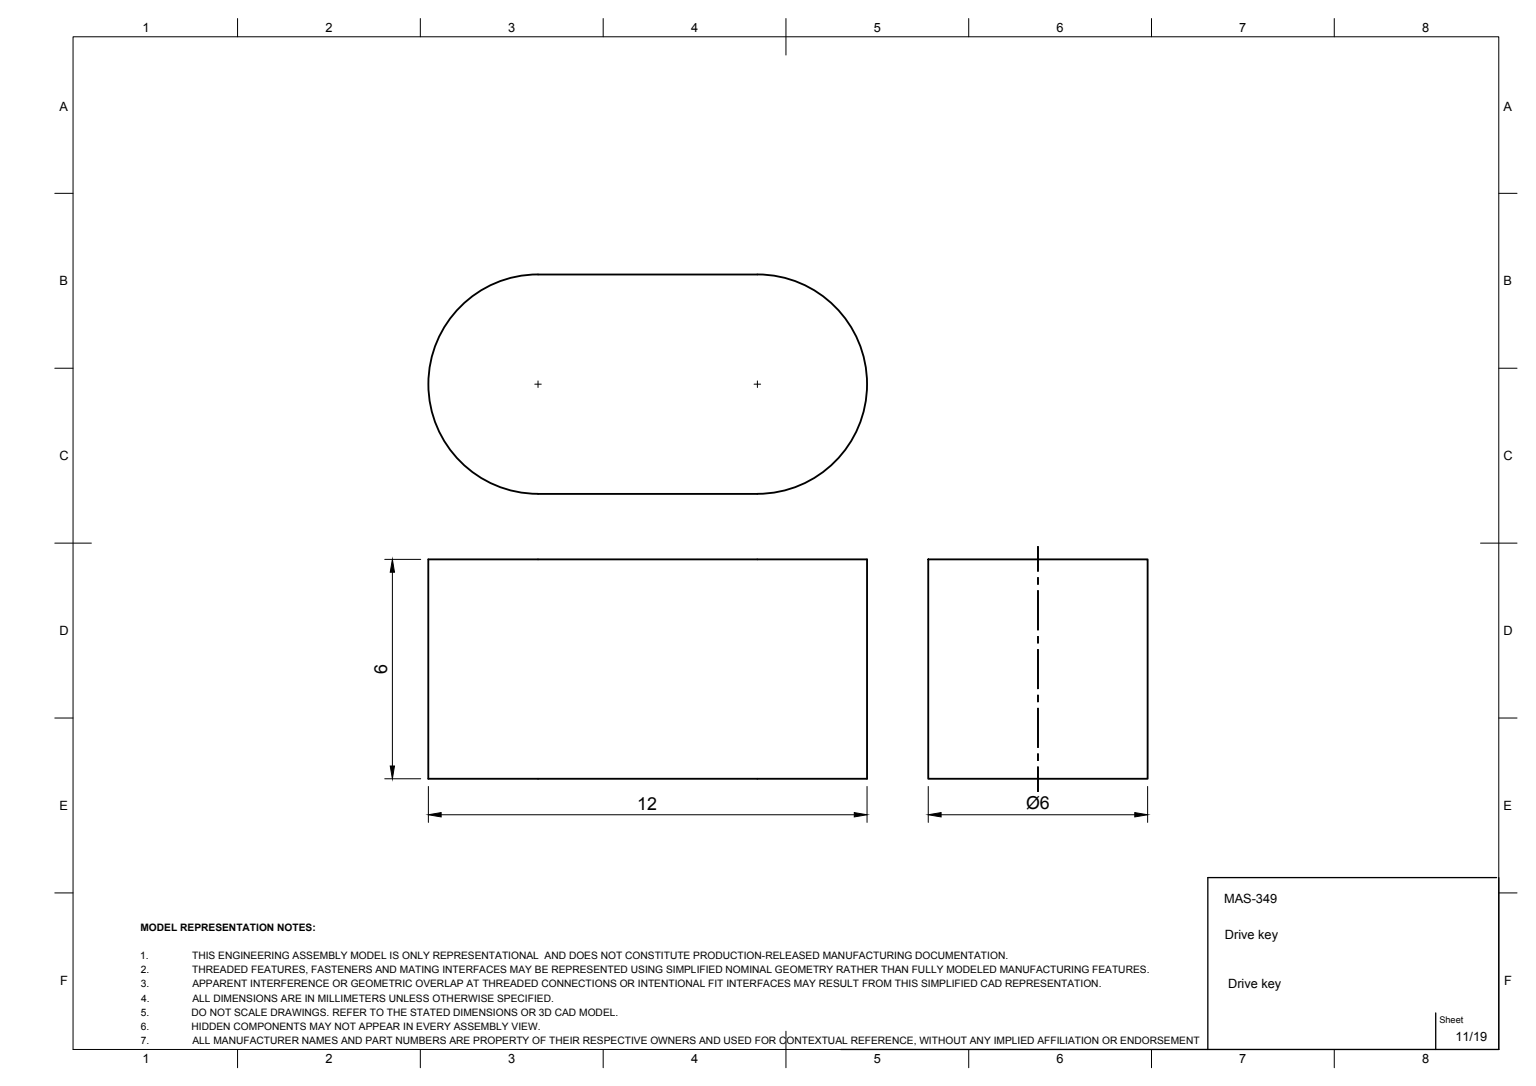
ISO-10303-21;
HEADER;
/* Generated by software containing ST-Developer
 * from STEP Tools, Inc. (www.steptools.com) 
 */

FILE_DESCRIPTION(
/* description */ ('Independent two-stage semi-open centrifugal-pump CAD. Shared impeller
s, open-machinable return casings, removable diaphragms, bronze wear/j
ournal rings, volume-preserving seal instances, retained keyed shaft, 
opposed mechanical face rings and partly threaded tie hardware. Native
 shaft rotation. Geometric topology/clearance only; flow/head/efficien
cy, pressure, cavitation, balance, preload, face loading and secondary
 seal fits/bonds, material/thermal/tolerance selection and life unassi
gned. External drive, coupling, anchors and piping bolts omitted.'),
/* implementation_level */ '2;1');

FILE_NAME(
/* name */ 'Drive key.step',
/* time_stamp */ '2026-11-08T18:06:32-08:00',
/* author */ (''),
/* organization */ (''),
/* preprocessor_version */ 'ST-DEVELOPER v20.2',
/* originating_system */ 'Autodesk Translation Framework v15.17.0.0',
/* authorisation */ '');

FILE_SCHEMA (('AUTOMOTIVE_DESIGN { 1 0 10303 214 3 1 1 }'));
ENDSEC;

DATA;
#10=MECHANICAL_DESIGN_GEOMETRIC_PRESENTATION_REPRESENTATION('',(#405),#16687);
#367=SHAPE_REPRESENTATION_RELATIONSHIP('SRR','None',#16776,#386);
#386=ADVANCED_BREP_SHAPE_REPRESENTATION('',(#424),#16680);
#405=STYLED_ITEM('',(#16876),#424);
#424=MANIFOLD_SOLID_BREP('Body1',#6124);
#659=PLANE('',#6861);
#660=PLANE('',#6865);
#661=PLANE('',#6869);
#662=PLANE('',#6870);
#974=FACE_OUTER_BOUND('',#1433,.T.);
#975=FACE_OUTER_BOUND('',#1434,.T.);
#976=FACE_OUTER_BOUND('',#1435,.T.);
#977=FACE_OUTER_BOUND('',#1436,.T.);
#978=FACE_OUTER_BOUND('',#1437,.T.);
#979=FACE_OUTER_BOUND('',#1438,.T.);
#1433=EDGE_LOOP('',(#5305,#5306,#5307,#5308));
#1434=EDGE_LOOP('',(#5309,#5310,#5311,#5312));
#1435=EDGE_LOOP('',(#5313,#5314,#5315,#5316));
#1436=EDGE_LOOP('',(#5317,#5318,#5319,#5320));
#1437=EDGE_LOOP('',(#5321,#5322,#5323,#5324));
#1438=EDGE_LOOP('',(#5325,#5326,#5327,#5328));
#1812=LINE('',#15164,#2181);
#1813=LINE('',#15166,#2182);
#1814=LINE('',#15168,#2183);
#1815=LINE('',#15169,#2184);
#1816=LINE('',#15175,#2185);
#1817=LINE('',#15178,#2186);
#1818=LINE('',#15180,#2187);
#1819=LINE('',#15181,#2188);
#2181=VECTOR('',#8340,1.);
#2182=VECTOR('',#8341,1.);
#2183=VECTOR('',#8342,1.);
#2184=VECTOR('',#8343,1.);
#2185=VECTOR('',#8350,1.);
#2186=VECTOR('',#8353,1.);
#2187=VECTOR('',#8354,1.);
#2188=VECTOR('',#8355,1.);
#2466=CIRCLE('',#6863,0.3);
#2467=CIRCLE('',#6864,0.3);
#2468=CIRCLE('',#6867,0.3);
#2469=CIRCLE('',#6868,0.3);
#2969=VERTEX_POINT('',#15162);
#2970=VERTEX_POINT('',#15163);
#2971=VERTEX_POINT('',#15165);
#2972=VERTEX_POINT('',#15167);
#2973=VERTEX_POINT('',#15171);
#2974=VERTEX_POINT('',#15173);
#2975=VERTEX_POINT('',#15177);
#2976=VERTEX_POINT('',#15179);
#3762=EDGE_CURVE('',#2969,#2970,#1812,.T.);
#3763=EDGE_CURVE('',#2969,#2971,#1813,.T.);
#3764=EDGE_CURVE('',#2972,#2971,#1814,.T.);
#3765=EDGE_CURVE('',#2970,#2972,#1815,.T.);
#3766=EDGE_CURVE('',#2973,#2970,#2466,.T.);
#3767=EDGE_CURVE('',#2974,#2972,#2467,.T.);
#3768=EDGE_CURVE('',#2973,#2974,#1816,.T.);
#3769=EDGE_CURVE('',#2973,#2975,#1817,.T.);
#3770=EDGE_CURVE('',#2976,#2974,#1818,.T.);
#3771=EDGE_CURVE('',#2975,#2976,#1819,.T.);
#3772=EDGE_CURVE('',#2969,#2975,#2468,.T.);
#3773=EDGE_CURVE('',#2971,#2976,#2469,.T.);
#5305=ORIENTED_EDGE('',*,*,#3762,.F.);
#5306=ORIENTED_EDGE('',*,*,#3763,.T.);
#5307=ORIENTED_EDGE('',*,*,#3764,.F.);
#5308=ORIENTED_EDGE('',*,*,#3765,.F.);
#5309=ORIENTED_EDGE('',*,*,#3766,.T.);
#5310=ORIENTED_EDGE('',*,*,#3765,.T.);
#5311=ORIENTED_EDGE('',*,*,#3767,.F.);
#5312=ORIENTED_EDGE('',*,*,#3768,.F.);
#5313=ORIENTED_EDGE('',*,*,#3769,.F.);
#5314=ORIENTED_EDGE('',*,*,#3768,.T.);
#5315=ORIENTED_EDGE('',*,*,#3770,.F.);
#5316=ORIENTED_EDGE('',*,*,#3771,.F.);
#5317=ORIENTED_EDGE('',*,*,#3772,.T.);
#5318=ORIENTED_EDGE('',*,*,#3771,.T.);
#5319=ORIENTED_EDGE('',*,*,#3773,.F.);
#5320=ORIENTED_EDGE('',*,*,#3763,.F.);
#5321=ORIENTED_EDGE('',*,*,#3773,.T.);
#5322=ORIENTED_EDGE('',*,*,#3770,.T.);
#5323=ORIENTED_EDGE('',*,*,#3767,.T.);
#5324=ORIENTED_EDGE('',*,*,#3764,.T.);
#5325=ORIENTED_EDGE('',*,*,#3772,.F.);
#5326=ORIENTED_EDGE('',*,*,#3762,.T.);
#5327=ORIENTED_EDGE('',*,*,#3766,.F.);
#5328=ORIENTED_EDGE('',*,*,#3769,.T.);
#5736=CYLINDRICAL_SURFACE('',#6862,0.3);
#5737=CYLINDRICAL_SURFACE('',#6866,0.3);
#6053=ADVANCED_FACE('',(#974),#659,.T.);
#6054=ADVANCED_FACE('',(#975),#5736,.T.);
#6055=ADVANCED_FACE('',(#976),#660,.T.);
#6056=ADVANCED_FACE('',(#977),#5737,.T.);
#6057=ADVANCED_FACE('',(#978),#661,.T.);
#6058=ADVANCED_FACE('',(#979),#662,.F.);
#6124=CLOSED_SHELL('',(#6053,#6054,#6055,#6056,#6057,#6058));
#6860=AXIS2_PLACEMENT_3D('',#15160,#8336,#8337);
#6861=AXIS2_PLACEMENT_3D('',#15161,#8338,#8339);
#6862=AXIS2_PLACEMENT_3D('',#15170,#8344,#8345);
#6863=AXIS2_PLACEMENT_3D('',#15172,#8346,#8347);
#6864=AXIS2_PLACEMENT_3D('',#15174,#8348,#8349);
#6865=AXIS2_PLACEMENT_3D('',#15176,#8351,#8352);
#6866=AXIS2_PLACEMENT_3D('',#15182,#8356,#8357);
#6867=AXIS2_PLACEMENT_3D('',#15183,#8358,#8359);
#6868=AXIS2_PLACEMENT_3D('',#15184,#8360,#8361);
#6869=AXIS2_PLACEMENT_3D('',#15185,#8362,#8363);
#6870=AXIS2_PLACEMENT_3D('',#15186,#8364,#8365);
#8336=DIRECTION('axis',(0.,0.,1.));
#8337=DIRECTION('refdir',(1.,0.,0.));
#8338=DIRECTION('center_axis',(0.,1.,0.));
#8339=DIRECTION('ref_axis',(0.,0.,1.));
#8340=DIRECTION('',(0.,0.,-1.));
#8341=DIRECTION('',(1.,0.,0.));
#8342=DIRECTION('',(0.,0.,1.));
#8343=DIRECTION('',(1.,0.,0.));
#8344=DIRECTION('center_axis',(1.,0.,0.));
#8345=DIRECTION('ref_axis',(0.,-1.,0.));
#8346=DIRECTION('center_axis',(1.,0.,0.));
#8347=DIRECTION('ref_axis',(0.,-1.,0.));
#8348=DIRECTION('center_axis',(1.,0.,0.));
#8349=DIRECTION('ref_axis',(0.,-1.,0.));
#8350=DIRECTION('',(1.,0.,0.));
#8351=DIRECTION('center_axis',(0.,-1.,0.));
#8352=DIRECTION('ref_axis',(0.,0.,-1.));
#8353=DIRECTION('',(0.,0.,1.));
#8354=DIRECTION('',(0.,0.,-1.));
#8355=DIRECTION('',(1.,0.,0.));
#8356=DIRECTION('center_axis',(1.,0.,0.));
#8357=DIRECTION('ref_axis',(0.,1.,0.));
#8358=DIRECTION('center_axis',(1.,0.,0.));
#8359=DIRECTION('ref_axis',(0.,1.,0.));
#8360=DIRECTION('center_axis',(1.,0.,0.));
#8361=DIRECTION('ref_axis',(0.,1.,0.));
#8362=DIRECTION('center_axis',(1.,0.,0.));
#8363=DIRECTION('ref_axis',(0.,0.,-1.));
#8364=DIRECTION('center_axis',(1.,0.,0.));
#8365=DIRECTION('ref_axis',(0.,0.,-1.));
#15160=CARTESIAN_POINT('',(0.,0.,0.));
#15161=CARTESIAN_POINT('Origin',(0.,0.3,2.1));
#15162=CARTESIAN_POINT('',(0.,0.3,2.7));
#15163=CARTESIAN_POINT('',(0.,0.3,2.1));
#15164=CARTESIAN_POINT('',(0.,0.3,2.7));
#15165=CARTESIAN_POINT('',(0.6,0.3,2.7));
#15166=CARTESIAN_POINT('',(0.,0.3,2.7));
#15167=CARTESIAN_POINT('',(0.6,0.3,2.1));
#15168=CARTESIAN_POINT('',(0.6,0.3,2.7));
#15169=CARTESIAN_POINT('',(0.,0.3,2.1));
#15170=CARTESIAN_POINT('Origin',(0.,0.,2.1));
#15171=CARTESIAN_POINT('',(0.,-0.3,2.1));
#15172=CARTESIAN_POINT('Origin',(0.,0.,2.1));
#15173=CARTESIAN_POINT('',(0.6,-0.3,2.1));
#15174=CARTESIAN_POINT('Origin',(0.6,0.,2.1));
#15175=CARTESIAN_POINT('',(0.,-0.3,2.1));
#15176=CARTESIAN_POINT('Origin',(0.,-0.3,2.7));
#15177=CARTESIAN_POINT('',(0.,-0.3,2.7));
#15178=CARTESIAN_POINT('',(0.,-0.3,2.1));
#15179=CARTESIAN_POINT('',(0.6,-0.3,2.7));
#15180=CARTESIAN_POINT('',(0.6,-0.3,2.1));
#15181=CARTESIAN_POINT('',(0.,-0.3,2.7));
#15182=CARTESIAN_POINT('Origin',(0.,2.77555756156289E-17,2.7));
#15183=CARTESIAN_POINT('Origin',(0.,2.77555756156289E-17,2.7));
#15184=CARTESIAN_POINT('Origin',(0.6,2.77555756156289E-17,2.7));
#15185=CARTESIAN_POINT('Origin',(0.6,0.,2.4));
#15186=CARTESIAN_POINT('Origin',(0.,0.,2.4));
#16659=UNCERTAINTY_MEASURE_WITH_UNIT(LENGTH_MEASURE(0.001),#16688,
'DISTANCE_ACCURACY_VALUE',
'Maximum model space distance between geometric entities at asserted c
onnectivities');
#16666=UNCERTAINTY_MEASURE_WITH_UNIT(LENGTH_MEASURE(0.001),#16688,
'DISTANCE_ACCURACY_VALUE',
'Maximum model space distance between geometric entities at asserted c
onnectivities');
#16680=(
GEOMETRIC_REPRESENTATION_CONTEXT(3)
GLOBAL_UNCERTAINTY_ASSIGNED_CONTEXT((#16659))
GLOBAL_UNIT_ASSIGNED_CONTEXT((#16688,#16690,#16691))
REPRESENTATION_CONTEXT('','3D')
);
#16687=(
GEOMETRIC_REPRESENTATION_CONTEXT(3)
GLOBAL_UNCERTAINTY_ASSIGNED_CONTEXT((#16666))
GLOBAL_UNIT_ASSIGNED_CONTEXT((#16688,#16690,#16691))
REPRESENTATION_CONTEXT('','3D')
);
#16688=(
LENGTH_UNIT()
NAMED_UNIT(*)
SI_UNIT(.CENTI.,.METRE.)
);
#16690=(
NAMED_UNIT(*)
PLANE_ANGLE_UNIT()
SI_UNIT($,.RADIAN.)
);
#16691=(
NAMED_UNIT(*)
SI_UNIT($,.STERADIAN.)
SOLID_ANGLE_UNIT()
);
#16705=SHAPE_DEFINITION_REPRESENTATION(#16725,#16776);
#16725=PRODUCT_DEFINITION_SHAPE('',$,#16797);
#16776=SHAPE_REPRESENTATION('',(#6860),#16680);
#16783=PRODUCT_DEFINITION_CONTEXT('part definition',#16845,'design');
#16797=PRODUCT_DEFINITION('Drive key','Drive key',#16817,#16783);
#16817=PRODUCT_DEFINITION_FORMATION('',$,#16860);
#16845=APPLICATION_CONTEXT(
'Core Data for Automotive Mechanical Design Process');
#16846=PRODUCT_CONTEXT('part definition',#16845,'mechanical');
#16860=PRODUCT('Drive key','Drive key',$,(#16846));
#16876=PRESENTATION_STYLE_ASSIGNMENT((#16891));
#16891=SURFACE_STYLE_USAGE(.BOTH.,#16906);
#16906=SURFACE_SIDE_STYLE('',(#16921));
#16921=SURFACE_STYLE_FILL_AREA(#16936);
#16936=FILL_AREA_STYLE('Key gray',(#16951));
#16951=FILL_AREA_STYLE_COLOUR('Key gray',#16966);
#16966=COLOUR_RGB('Key gray',0.725490196078431,0.752941176470588,0.792156862745098);
ENDSEC;
END-ISO-10303-21;
